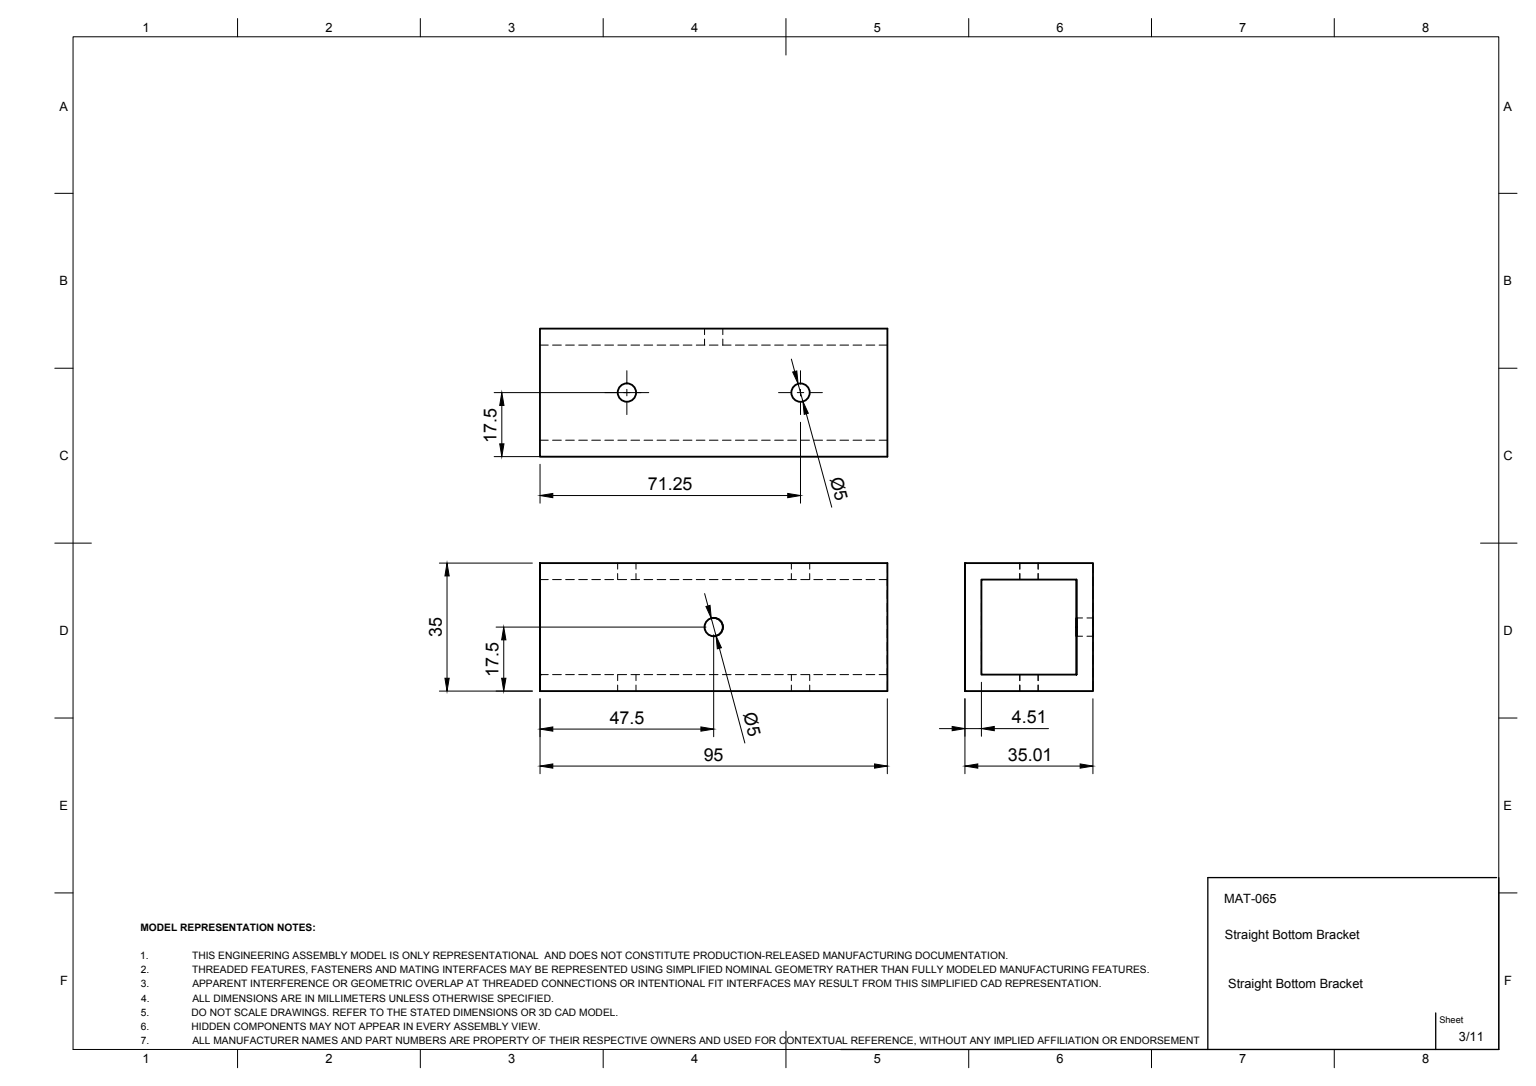
ISO-10303-21;
HEADER;
/* Generated by software containing ST-Developer
 * from STEP Tools, Inc. (www.steptools.com) 
 */

FILE_DESCRIPTION(
/* description */ (
'CAx-IF Rec.Pracs.---Representation and Presentation of Product Manufa
cturing Information (PMI)---4.0---2014-10-13'),
/* implementation_level */ '2;1');

FILE_NAME(
/* name */ 'Straight Bottom Bracket.step',
/* time_stamp */ '2026-11-15T23:28:27-08:00',
/* author */ (''),
/* organization */ (''),
/* preprocessor_version */ 'ST-DEVELOPER v20.2',
/* originating_system */ 'Autodesk Translation Framework v15.17.0.0',
/* authorisation */ '');

FILE_SCHEMA (('AUTOMOTIVE_DESIGN { 1 0 10303 214 3 1 1 }'));
ENDSEC;

DATA;
#10=MECHANICAL_DESIGN_GEOMETRIC_PRESENTATION_REPRESENTATION('',(#189),#7756);
#171=SHAPE_REPRESENTATION_RELATIONSHIP('SRR','None',#7819,#180);
#180=ADVANCED_BREP_SHAPE_REPRESENTATION('',(#198),#7747);
#189=STYLED_ITEM('',(#7873),#198);
#198=MANIFOLD_SOLID_BREP('Body1',#4626);
#207=CYLINDRICAL_SURFACE('',#4757,0.0025);
#208=CYLINDRICAL_SURFACE('',#4758,0.0025);
#209=CYLINDRICAL_SURFACE('',#4759,0.0025);
#210=CYLINDRICAL_SURFACE('',#4760,0.0025);
#211=CYLINDRICAL_SURFACE('',#4761,0.0025);
#264=CIRCLE('',#4740,0.0025);
#265=CIRCLE('',#4743,0.0025);
#266=CIRCLE('',#4744,0.0025);
#267=CIRCLE('',#4746,0.0025);
#268=CIRCLE('',#4747,0.0025);
#269=CIRCLE('',#4749,0.0025);
#270=CIRCLE('',#4750,0.0025);
#271=CIRCLE('',#4752,0.0025);
#272=CIRCLE('',#4754,0.0025);
#273=CIRCLE('',#4755,0.0025);
#378=FACE_BOUND('',#686,.T.);
#379=FACE_BOUND('',#688,.T.);
#380=FACE_BOUND('',#690,.T.);
#381=FACE_BOUND('',#693,.T.);
#382=FACE_BOUND('',#694,.T.);
#383=FACE_BOUND('',#696,.T.);
#384=FACE_BOUND('',#697,.T.);
#385=FACE_BOUND('',#699,.T.);
#386=FACE_BOUND('',#700,.T.);
#387=FACE_BOUND('',#702,.T.);
#388=FACE_BOUND('',#704,.T.);
#389=FACE_BOUND('',#705,.T.);
#452=FACE_OUTER_BOUND('',#685,.T.);
#453=FACE_OUTER_BOUND('',#687,.T.);
#454=FACE_OUTER_BOUND('',#689,.T.);
#455=FACE_OUTER_BOUND('',#691,.T.);
#456=FACE_OUTER_BOUND('',#692,.T.);
#457=FACE_OUTER_BOUND('',#695,.T.);
#458=FACE_OUTER_BOUND('',#698,.T.);
#459=FACE_OUTER_BOUND('',#701,.T.);
#460=FACE_OUTER_BOUND('',#703,.T.);
#461=FACE_OUTER_BOUND('',#706,.T.);
#462=FACE_OUTER_BOUND('',#707,.T.);
#463=FACE_OUTER_BOUND('',#708,.T.);
#464=FACE_OUTER_BOUND('',#709,.T.);
#465=FACE_OUTER_BOUND('',#710,.T.);
#466=FACE_OUTER_BOUND('',#711,.T.);
#685=EDGE_LOOP('',(#2993,#2994,#2995,#2996));
#686=EDGE_LOOP('',(#2997,#2998,#2999,#3000));
#687=EDGE_LOOP('',(#3001,#3002,#3003,#3004));
#688=EDGE_LOOP('',(#3005,#3006,#3007,#3008));
#689=EDGE_LOOP('',(#3009,#3010,#3011,#3012));
#690=EDGE_LOOP('',(#3013));
#691=EDGE_LOOP('',(#3014,#3015,#3016,#3017));
#692=EDGE_LOOP('',(#3018,#3019,#3020,#3021));
#693=EDGE_LOOP('',(#3022));
#694=EDGE_LOOP('',(#3023));
#695=EDGE_LOOP('',(#3024,#3025,#3026,#3027));
#696=EDGE_LOOP('',(#3028));
#697=EDGE_LOOP('',(#3029));
#698=EDGE_LOOP('',(#3030,#3031,#3032,#3033));
#699=EDGE_LOOP('',(#3034));
#700=EDGE_LOOP('',(#3035));
#701=EDGE_LOOP('',(#3036,#3037,#3038,#3039));
#702=EDGE_LOOP('',(#3040));
#703=EDGE_LOOP('',(#3041,#3042,#3043,#3044));
#704=EDGE_LOOP('',(#3045));
#705=EDGE_LOOP('',(#3046));
#706=EDGE_LOOP('',(#3047,#3048,#3049,#3050));
#707=EDGE_LOOP('',(#3051,#3052,#3053,#3054));
#708=EDGE_LOOP('',(#3055,#3056,#3057,#3058));
#709=EDGE_LOOP('',(#3059,#3060,#3061,#3062));
#710=EDGE_LOOP('',(#3063,#3064,#3065,#3066));
#711=EDGE_LOOP('',(#3067,#3068,#3069,#3070));
#992=LINE('',#6424,#1485);
#993=LINE('',#6426,#1486);
#994=LINE('',#6428,#1487);
#995=LINE('',#6429,#1488);
#996=LINE('',#6432,#1489);
#997=LINE('',#6434,#1490);
#998=LINE('',#6436,#1491);
#999=LINE('',#6437,#1492);
#1000=LINE('',#6441,#1493);
#1001=LINE('',#6443,#1494);
#1002=LINE('',#6445,#1495);
#1003=LINE('',#6446,#1496);
#1004=LINE('',#6449,#1497);
#1005=LINE('',#6451,#1498);
#1006=LINE('',#6453,#1499);
#1007=LINE('',#6454,#1500);
#1008=LINE('',#6456,#1501);
#1009=LINE('',#6457,#1502);
#1010=LINE('',#6461,#1503);
#1011=LINE('',#6462,#1504);
#1012=LINE('',#6474,#1505);
#1013=LINE('',#6475,#1506);
#1014=LINE('',#6481,#1507);
#1015=LINE('',#6485,#1508);
#1016=LINE('',#6492,#1509);
#1017=LINE('',#6494,#1510);
#1018=LINE('',#6496,#1511);
#1019=LINE('',#6498,#1512);
#1020=LINE('',#6500,#1513);
#1485=VECTOR('',#5138,1.);
#1486=VECTOR('',#5139,1.);
#1487=VECTOR('',#5140,1.);
#1488=VECTOR('',#5141,1.);
#1489=VECTOR('',#5142,1.);
#1490=VECTOR('',#5143,1.);
#1491=VECTOR('',#5144,1.);
#1492=VECTOR('',#5145,1.);
#1493=VECTOR('',#5148,1.);
#1494=VECTOR('',#5149,1.);
#1495=VECTOR('',#5150,1.);
#1496=VECTOR('',#5151,1.);
#1497=VECTOR('',#5152,1.);
#1498=VECTOR('',#5153,1.);
#1499=VECTOR('',#5154,1.);
#1500=VECTOR('',#5155,1.);
#1501=VECTOR('',#5158,1.);
#1502=VECTOR('',#5159,1.);
#1503=VECTOR('',#5164,1.);
#1504=VECTOR('',#5165,1.);
#1505=VECTOR('',#5180,1.);
#1506=VECTOR('',#5181,1.);
#1507=VECTOR('',#5188,1.);
#1508=VECTOR('',#5193,1.);
#1509=VECTOR('',#5202,0.0025);
#1510=VECTOR('',#5205,0.0025);
#1511=VECTOR('',#5208,0.0025);
#1512=VECTOR('',#5211,0.0025);
#1513=VECTOR('',#5214,0.0025);
#1978=VERTEX_POINT('',#6422);
#1979=VERTEX_POINT('',#6423);
#1980=VERTEX_POINT('',#6425);
#1981=VERTEX_POINT('',#6427);
#1982=VERTEX_POINT('',#6430);
#1983=VERTEX_POINT('',#6431);
#1984=VERTEX_POINT('',#6433);
#1985=VERTEX_POINT('',#6435);
#1986=VERTEX_POINT('',#6439);
#1987=VERTEX_POINT('',#6440);
#1988=VERTEX_POINT('',#6442);
#1989=VERTEX_POINT('',#6444);
#1990=VERTEX_POINT('',#6447);
#1991=VERTEX_POINT('',#6448);
#1992=VERTEX_POINT('',#6450);
#1993=VERTEX_POINT('',#6452);
#1994=VERTEX_POINT('',#6458);
#1995=VERTEX_POINT('',#6464);
#1996=VERTEX_POINT('',#6466);
#1997=VERTEX_POINT('',#6469);
#1998=VERTEX_POINT('',#6471);
#1999=VERTEX_POINT('',#6476);
#2000=VERTEX_POINT('',#6478);
#2001=VERTEX_POINT('',#6482);
#2002=VERTEX_POINT('',#6486);
#2003=VERTEX_POINT('',#6488);
#2380=EDGE_CURVE('',#1978,#1979,#992,.T.);
#2381=EDGE_CURVE('',#1980,#1979,#993,.T.);
#2382=EDGE_CURVE('',#1981,#1980,#994,.T.);
#2383=EDGE_CURVE('',#1981,#1978,#995,.T.);
#2384=EDGE_CURVE('',#1982,#1983,#996,.T.);
#2385=EDGE_CURVE('',#1983,#1984,#997,.T.);
#2386=EDGE_CURVE('',#1985,#1984,#998,.T.);
#2387=EDGE_CURVE('',#1982,#1985,#999,.T.);
#2388=EDGE_CURVE('',#1986,#1987,#1000,.T.);
#2389=EDGE_CURVE('',#1988,#1986,#1001,.T.);
#2390=EDGE_CURVE('',#1988,#1989,#1002,.T.);
#2391=EDGE_CURVE('',#1989,#1987,#1003,.T.);
#2392=EDGE_CURVE('',#1990,#1991,#1004,.T.);
#2393=EDGE_CURVE('',#1991,#1992,#1005,.T.);
#2394=EDGE_CURVE('',#1993,#1992,#1006,.T.);
#2395=EDGE_CURVE('',#1990,#1993,#1007,.T.);
#2396=EDGE_CURVE('',#1978,#1986,#1008,.T.);
#2397=EDGE_CURVE('',#1981,#1988,#1009,.T.);
#2398=EDGE_CURVE('',#1994,#1994,#264,.T.);
#2399=EDGE_CURVE('',#1979,#1987,#1010,.T.);
#2400=EDGE_CURVE('',#1980,#1989,#1011,.T.);
#2401=EDGE_CURVE('',#1995,#1995,#265,.T.);
#2402=EDGE_CURVE('',#1996,#1996,#266,.T.);
#2403=EDGE_CURVE('',#1997,#1997,#267,.T.);
#2404=EDGE_CURVE('',#1998,#1998,#268,.T.);
#2405=EDGE_CURVE('',#1991,#1983,#1012,.T.);
#2406=EDGE_CURVE('',#1992,#1982,#1013,.T.);
#2407=EDGE_CURVE('',#1999,#1999,#269,.T.);
#2408=EDGE_CURVE('',#2000,#2000,#270,.T.);
#2409=EDGE_CURVE('',#1993,#1985,#1014,.T.);
#2410=EDGE_CURVE('',#2001,#2001,#271,.T.);
#2411=EDGE_CURVE('',#1990,#1984,#1015,.T.);
#2412=EDGE_CURVE('',#2002,#2002,#272,.T.);
#2413=EDGE_CURVE('',#2003,#2003,#273,.T.);
#2414=EDGE_CURVE('',#2001,#1994,#1016,.T.);
#2415=EDGE_CURVE('',#1998,#2003,#1017,.T.);
#2416=EDGE_CURVE('',#1997,#2002,#1018,.T.);
#2417=EDGE_CURVE('',#2000,#1996,#1019,.T.);
#2418=EDGE_CURVE('',#1999,#1995,#1020,.T.);
#2993=ORIENTED_EDGE('',*,*,#2380,.T.);
#2994=ORIENTED_EDGE('',*,*,#2381,.F.);
#2995=ORIENTED_EDGE('',*,*,#2382,.F.);
#2996=ORIENTED_EDGE('',*,*,#2383,.T.);
#2997=ORIENTED_EDGE('',*,*,#2384,.T.);
#2998=ORIENTED_EDGE('',*,*,#2385,.T.);
#2999=ORIENTED_EDGE('',*,*,#2386,.F.);
#3000=ORIENTED_EDGE('',*,*,#2387,.F.);
#3001=ORIENTED_EDGE('',*,*,#2388,.F.);
#3002=ORIENTED_EDGE('',*,*,#2389,.F.);
#3003=ORIENTED_EDGE('',*,*,#2390,.T.);
#3004=ORIENTED_EDGE('',*,*,#2391,.T.);
#3005=ORIENTED_EDGE('',*,*,#2392,.T.);
#3006=ORIENTED_EDGE('',*,*,#2393,.T.);
#3007=ORIENTED_EDGE('',*,*,#2394,.F.);
#3008=ORIENTED_EDGE('',*,*,#2395,.F.);
#3009=ORIENTED_EDGE('',*,*,#2396,.F.);
#3010=ORIENTED_EDGE('',*,*,#2383,.F.);
#3011=ORIENTED_EDGE('',*,*,#2397,.T.);
#3012=ORIENTED_EDGE('',*,*,#2389,.T.);
#3013=ORIENTED_EDGE('',*,*,#2398,.F.);
#3014=ORIENTED_EDGE('',*,*,#2399,.T.);
#3015=ORIENTED_EDGE('',*,*,#2391,.F.);
#3016=ORIENTED_EDGE('',*,*,#2400,.F.);
#3017=ORIENTED_EDGE('',*,*,#2381,.T.);
#3018=ORIENTED_EDGE('',*,*,#2397,.F.);
#3019=ORIENTED_EDGE('',*,*,#2382,.T.);
#3020=ORIENTED_EDGE('',*,*,#2400,.T.);
#3021=ORIENTED_EDGE('',*,*,#2390,.F.);
#3022=ORIENTED_EDGE('',*,*,#2401,.F.);
#3023=ORIENTED_EDGE('',*,*,#2402,.F.);
#3024=ORIENTED_EDGE('',*,*,#2396,.T.);
#3025=ORIENTED_EDGE('',*,*,#2388,.T.);
#3026=ORIENTED_EDGE('',*,*,#2399,.F.);
#3027=ORIENTED_EDGE('',*,*,#2380,.F.);
#3028=ORIENTED_EDGE('',*,*,#2403,.T.);
#3029=ORIENTED_EDGE('',*,*,#2404,.T.);
#3030=ORIENTED_EDGE('',*,*,#2405,.T.);
#3031=ORIENTED_EDGE('',*,*,#2384,.F.);
#3032=ORIENTED_EDGE('',*,*,#2406,.F.);
#3033=ORIENTED_EDGE('',*,*,#2393,.F.);
#3034=ORIENTED_EDGE('',*,*,#2407,.F.);
#3035=ORIENTED_EDGE('',*,*,#2408,.F.);
#3036=ORIENTED_EDGE('',*,*,#2394,.T.);
#3037=ORIENTED_EDGE('',*,*,#2406,.T.);
#3038=ORIENTED_EDGE('',*,*,#2387,.T.);
#3039=ORIENTED_EDGE('',*,*,#2409,.F.);
#3040=ORIENTED_EDGE('',*,*,#2410,.T.);
#3041=ORIENTED_EDGE('',*,*,#2395,.T.);
#3042=ORIENTED_EDGE('',*,*,#2409,.T.);
#3043=ORIENTED_EDGE('',*,*,#2386,.T.);
#3044=ORIENTED_EDGE('',*,*,#2411,.F.);
#3045=ORIENTED_EDGE('',*,*,#2412,.T.);
#3046=ORIENTED_EDGE('',*,*,#2413,.T.);
#3047=ORIENTED_EDGE('',*,*,#2411,.T.);
#3048=ORIENTED_EDGE('',*,*,#2385,.F.);
#3049=ORIENTED_EDGE('',*,*,#2405,.F.);
#3050=ORIENTED_EDGE('',*,*,#2392,.F.);
#3051=ORIENTED_EDGE('',*,*,#2410,.F.);
#3052=ORIENTED_EDGE('',*,*,#2414,.T.);
#3053=ORIENTED_EDGE('',*,*,#2398,.T.);
#3054=ORIENTED_EDGE('',*,*,#2414,.F.);
#3055=ORIENTED_EDGE('',*,*,#2404,.F.);
#3056=ORIENTED_EDGE('',*,*,#2415,.T.);
#3057=ORIENTED_EDGE('',*,*,#2413,.F.);
#3058=ORIENTED_EDGE('',*,*,#2415,.F.);
#3059=ORIENTED_EDGE('',*,*,#2403,.F.);
#3060=ORIENTED_EDGE('',*,*,#2416,.T.);
#3061=ORIENTED_EDGE('',*,*,#2412,.F.);
#3062=ORIENTED_EDGE('',*,*,#2416,.F.);
#3063=ORIENTED_EDGE('',*,*,#2408,.T.);
#3064=ORIENTED_EDGE('',*,*,#2417,.T.);
#3065=ORIENTED_EDGE('',*,*,#2402,.T.);
#3066=ORIENTED_EDGE('',*,*,#2417,.F.);
#3067=ORIENTED_EDGE('',*,*,#2407,.T.);
#3068=ORIENTED_EDGE('',*,*,#2418,.T.);
#3069=ORIENTED_EDGE('',*,*,#2401,.T.);
#3070=ORIENTED_EDGE('',*,*,#2418,.F.);
#4219=PLANE('',#4737);
#4220=PLANE('',#4738);
#4221=PLANE('',#4739);
#4222=PLANE('',#4741);
#4223=PLANE('',#4742);
#4224=PLANE('',#4745);
#4225=PLANE('',#4748);
#4226=PLANE('',#4751);
#4227=PLANE('',#4753);
#4228=PLANE('',#4756);
#4393=ADVANCED_FACE('',(#452,#378),#4219,.F.);
#4394=ADVANCED_FACE('',(#453,#379),#4220,.T.);
#4395=ADVANCED_FACE('',(#454,#380),#4221,.T.);
#4396=ADVANCED_FACE('',(#455),#4222,.F.);
#4397=ADVANCED_FACE('',(#456,#381,#382),#4223,.T.);
#4398=ADVANCED_FACE('',(#457,#383,#384),#4224,.F.);
#4399=ADVANCED_FACE('',(#458,#385,#386),#4225,.T.);
#4400=ADVANCED_FACE('',(#459,#387),#4226,.F.);
#4401=ADVANCED_FACE('',(#460,#388,#389),#4227,.F.);
#4402=ADVANCED_FACE('',(#461),#4228,.T.);
#4403=ADVANCED_FACE('',(#462),#207,.F.);
#4404=ADVANCED_FACE('',(#463),#208,.F.);
#4405=ADVANCED_FACE('',(#464),#209,.F.);
#4406=ADVANCED_FACE('',(#465),#210,.F.);
#4407=ADVANCED_FACE('',(#466),#211,.F.);
#4626=CLOSED_SHELL('',(#4393,#4394,#4395,#4396,#4397,#4398,#4399,#4400,
#4401,#4402,#4403,#4404,#4405,#4406,#4407));
#4736=AXIS2_PLACEMENT_3D('',#6420,#5134,#5135);
#4737=AXIS2_PLACEMENT_3D('',#6421,#5136,#5137);
#4738=AXIS2_PLACEMENT_3D('',#6438,#5146,#5147);
#4739=AXIS2_PLACEMENT_3D('',#6455,#5156,#5157);
#4740=AXIS2_PLACEMENT_3D('',#6459,#5160,#5161);
#4741=AXIS2_PLACEMENT_3D('',#6460,#5162,#5163);
#4742=AXIS2_PLACEMENT_3D('',#6463,#5166,#5167);
#4743=AXIS2_PLACEMENT_3D('',#6465,#5168,#5169);
#4744=AXIS2_PLACEMENT_3D('',#6467,#5170,#5171);
#4745=AXIS2_PLACEMENT_3D('',#6468,#5172,#5173);
#4746=AXIS2_PLACEMENT_3D('',#6470,#5174,#5175);
#4747=AXIS2_PLACEMENT_3D('',#6472,#5176,#5177);
#4748=AXIS2_PLACEMENT_3D('',#6473,#5178,#5179);
#4749=AXIS2_PLACEMENT_3D('',#6477,#5182,#5183);
#4750=AXIS2_PLACEMENT_3D('',#6479,#5184,#5185);
#4751=AXIS2_PLACEMENT_3D('',#6480,#5186,#5187);
#4752=AXIS2_PLACEMENT_3D('',#6483,#5189,#5190);
#4753=AXIS2_PLACEMENT_3D('',#6484,#5191,#5192);
#4754=AXIS2_PLACEMENT_3D('',#6487,#5194,#5195);
#4755=AXIS2_PLACEMENT_3D('',#6489,#5196,#5197);
#4756=AXIS2_PLACEMENT_3D('',#6490,#5198,#5199);
#4757=AXIS2_PLACEMENT_3D('',#6491,#5200,#5201);
#4758=AXIS2_PLACEMENT_3D('',#6493,#5203,#5204);
#4759=AXIS2_PLACEMENT_3D('',#6495,#5206,#5207);
#4760=AXIS2_PLACEMENT_3D('',#6497,#5209,#5210);
#4761=AXIS2_PLACEMENT_3D('',#6499,#5212,#5213);
#5134=DIRECTION('axis',(0.,0.,1.));
#5135=DIRECTION('refdir',(1.,0.,0.));
#5136=DIRECTION('center_axis',(1.,0.,0.));
#5137=DIRECTION('ref_axis',(0.,0.,-1.));
#5138=DIRECTION('',(0.,-1.,0.));
#5139=DIRECTION('',(0.,0.,-1.));
#5140=DIRECTION('',(0.,-1.,0.));
#5141=DIRECTION('',(0.,0.,-1.));
#5142=DIRECTION('',(0.,-1.,0.));
#5143=DIRECTION('',(0.,0.,-1.));
#5144=DIRECTION('',(0.,-1.,0.));
#5145=DIRECTION('',(0.,-6.67201336914157E-17,-1.));
#5146=DIRECTION('center_axis',(1.,0.,0.));
#5147=DIRECTION('ref_axis',(0.,0.,-1.));
#5148=DIRECTION('',(0.,-1.,0.));
#5149=DIRECTION('',(0.,0.,-1.));
#5150=DIRECTION('',(0.,-1.,0.));
#5151=DIRECTION('',(0.,0.,-1.));
#5152=DIRECTION('',(0.,0.,1.));
#5153=DIRECTION('',(0.,1.,0.));
#5154=DIRECTION('',(0.,6.67201336914157E-17,1.));
#5155=DIRECTION('',(0.,1.,0.));
#5156=DIRECTION('center_axis',(-1.82602471155453E-16,1.,0.));
#5157=DIRECTION('ref_axis',(-1.,-1.82602471155453E-16,0.));
#5158=DIRECTION('',(1.,1.82602471155453E-16,0.));
#5159=DIRECTION('',(1.,1.82602471155453E-16,0.));
#5160=DIRECTION('center_axis',(-1.82602471155453E-16,1.,0.));
#5161=DIRECTION('ref_axis',(-1.,-1.82602471155453E-16,0.));
#5162=DIRECTION('center_axis',(-2.19122965386544E-16,1.,0.));
#5163=DIRECTION('ref_axis',(-1.,-2.19122965386544E-16,0.));
#5164=DIRECTION('',(1.,2.19122965386544E-16,0.));
#5165=DIRECTION('',(1.,2.19122965386544E-16,0.));
#5166=DIRECTION('center_axis',(0.,0.,1.));
#5167=DIRECTION('ref_axis',(1.,0.,0.));
#5168=DIRECTION('center_axis',(0.,0.,1.));
#5169=DIRECTION('ref_axis',(1.,0.,0.));
#5170=DIRECTION('center_axis',(0.,0.,1.));
#5171=DIRECTION('ref_axis',(1.,0.,0.));
#5172=DIRECTION('center_axis',(0.,0.,1.));
#5173=DIRECTION('ref_axis',(1.,0.,0.));
#5174=DIRECTION('center_axis',(0.,0.,1.));
#5175=DIRECTION('ref_axis',(1.,0.,0.));
#5176=DIRECTION('center_axis',(0.,0.,1.));
#5177=DIRECTION('ref_axis',(1.,0.,0.));
#5178=DIRECTION('center_axis',(0.,0.,-1.));
#5179=DIRECTION('ref_axis',(-1.,0.,0.));
#5180=DIRECTION('',(-1.,0.,0.));
#5181=DIRECTION('',(-1.,0.,0.));
#5182=DIRECTION('center_axis',(0.,0.,-1.));
#5183=DIRECTION('ref_axis',(-1.,0.,0.));
#5184=DIRECTION('center_axis',(0.,0.,-1.));
#5185=DIRECTION('ref_axis',(-1.,0.,0.));
#5186=DIRECTION('center_axis',(0.,1.,-6.67201336914157E-17));
#5187=DIRECTION('ref_axis',(0.,6.67201336914157E-17,1.));
#5188=DIRECTION('',(-1.,0.,0.));
#5189=DIRECTION('center_axis',(0.,1.,-6.67201336914157E-17));
#5190=DIRECTION('ref_axis',(0.,6.67201336914157E-17,1.));
#5191=DIRECTION('center_axis',(0.,0.,-1.));
#5192=DIRECTION('ref_axis',(-1.,0.,0.));
#5193=DIRECTION('',(-1.,0.,0.));
#5194=DIRECTION('center_axis',(0.,0.,-1.));
#5195=DIRECTION('ref_axis',(-1.,0.,0.));
#5196=DIRECTION('center_axis',(0.,0.,-1.));
#5197=DIRECTION('ref_axis',(-1.,0.,0.));
#5198=DIRECTION('center_axis',(0.,1.,0.));
#5199=DIRECTION('ref_axis',(0.,0.,1.));
#5200=DIRECTION('center_axis',(-1.82602471155453E-16,1.,0.));
#5201=DIRECTION('ref_axis',(-1.,-1.82602471155453E-16,0.));
#5202=DIRECTION('',(-1.82602471155453E-16,1.,0.));
#5203=DIRECTION('center_axis',(0.,0.,1.));
#5204=DIRECTION('ref_axis',(1.,0.,0.));
#5205=DIRECTION('',(0.,0.,1.));
#5206=DIRECTION('center_axis',(0.,0.,1.));
#5207=DIRECTION('ref_axis',(1.,0.,0.));
#5208=DIRECTION('',(0.,0.,1.));
#5209=DIRECTION('center_axis',(0.,0.,1.));
#5210=DIRECTION('ref_axis',(1.,0.,0.));
#5211=DIRECTION('',(0.,0.,1.));
#5212=DIRECTION('center_axis',(0.,0.,1.));
#5213=DIRECTION('ref_axis',(1.,0.,0.));
#5214=DIRECTION('',(0.,0.,1.));
#6420=CARTESIAN_POINT('',(0.,0.,0.));
#6421=CARTESIAN_POINT('Origin',(-0.0475,-1.04083408558608E-17,0.035));
#6422=CARTESIAN_POINT('',(-0.0475,0.0175,0.));
#6423=CARTESIAN_POINT('',(-0.0475,-0.0175,0.));
#6424=CARTESIAN_POINT('',(-0.0475,-1.04083408558608E-17,0.));
#6425=CARTESIAN_POINT('',(-0.0475,-0.0175,0.035));
#6426=CARTESIAN_POINT('',(-0.0475,-0.0175,0.035));
#6427=CARTESIAN_POINT('',(-0.0475,0.0175,0.035));
#6428=CARTESIAN_POINT('',(-0.0475,-1.04083408558608E-17,0.035));
#6429=CARTESIAN_POINT('',(-0.0475,0.0175,0.035));
#6430=CARTESIAN_POINT('',(-0.0475,0.013,0.0305));
#6431=CARTESIAN_POINT('',(-0.0475,-0.013,0.0305));
#6432=CARTESIAN_POINT('',(-0.0475,-1.04083408558608E-17,0.0305));
#6433=CARTESIAN_POINT('',(-0.0475,-0.013,0.0045));
#6434=CARTESIAN_POINT('',(-0.0475,-0.013,0.0175));
#6435=CARTESIAN_POINT('',(-0.0475,0.013,0.0045));
#6436=CARTESIAN_POINT('',(-0.0475,-1.21430643318376E-17,0.0045));
#6437=CARTESIAN_POINT('',(-0.0475,0.013,0.0175));
#6438=CARTESIAN_POINT('Origin',(0.0475,6.93889390390723E-18,0.035));
#6439=CARTESIAN_POINT('',(0.0475,0.0175,0.));
#6440=CARTESIAN_POINT('',(0.0475,-0.0175,0.));
#6441=CARTESIAN_POINT('',(0.0475,6.93889390390723E-18,0.));
#6442=CARTESIAN_POINT('',(0.0475,0.0175,0.035));
#6443=CARTESIAN_POINT('',(0.0475,0.0175,0.035));
#6444=CARTESIAN_POINT('',(0.0475,-0.0175,0.035));
#6445=CARTESIAN_POINT('',(0.0475,6.93889390390723E-18,0.035));
#6446=CARTESIAN_POINT('',(0.0475,-0.0175,0.035));
#6447=CARTESIAN_POINT('',(0.0475,-0.013,0.0045));
#6448=CARTESIAN_POINT('',(0.0475,-0.013,0.0305));
#6449=CARTESIAN_POINT('',(0.0475,-0.013,0.035));
#6450=CARTESIAN_POINT('',(0.0475,0.013,0.0305));
#6451=CARTESIAN_POINT('',(0.0475,6.93889390390723E-18,0.0305));
#6452=CARTESIAN_POINT('',(0.0475,0.013,0.0045));
#6453=CARTESIAN_POINT('',(0.0475,0.013,0.035));
#6454=CARTESIAN_POINT('',(0.0475,6.93889390390723E-18,0.0045));
#6455=CARTESIAN_POINT('Origin',(6.93889390390723E-18,0.0175,0.035));
#6456=CARTESIAN_POINT('',(6.93889390390723E-18,0.0175,0.));
#6457=CARTESIAN_POINT('',(6.93889390390723E-18,0.0175,0.035));
#6458=CARTESIAN_POINT('',(0.0025,0.0175,0.0175));
#6459=CARTESIAN_POINT('Origin',(-3.46944695195361E-18,0.0175,0.0175));
#6460=CARTESIAN_POINT('Origin',(6.93889390390723E-18,-0.0175,0.035));
#6461=CARTESIAN_POINT('',(6.93889390390723E-18,-0.0175,0.));
#6462=CARTESIAN_POINT('',(6.93889390390723E-18,-0.0175,0.035));
#6463=CARTESIAN_POINT('Origin',(6.93889390390723E-18,0.,0.035));
#6464=CARTESIAN_POINT('',(-0.02625,-1.53080849893419E-19,0.035));
#6465=CARTESIAN_POINT('Origin',(-0.02375,1.53080849893419E-19,0.035));
#6466=CARTESIAN_POINT('',(0.02125,-3.08148791101958E-34,0.035));
#6467=CARTESIAN_POINT('Origin',(0.02375,3.06161699786838E-19,0.035));
#6468=CARTESIAN_POINT('Origin',(6.93889390390723E-18,0.,0.));
#6469=CARTESIAN_POINT('',(-0.02625,-1.53080849893419E-19,0.));
#6470=CARTESIAN_POINT('Origin',(-0.02375,1.53080849893419E-19,0.));
#6471=CARTESIAN_POINT('',(0.02125,-3.08148791101958E-34,0.));
#6472=CARTESIAN_POINT('Origin',(0.02375,3.06161699786838E-19,0.));
#6473=CARTESIAN_POINT('Origin',(0.0525,-1.04083408558608E-17,0.0305));
#6474=CARTESIAN_POINT('',(0.0525,-0.013,0.0305));
#6475=CARTESIAN_POINT('',(0.0525,0.013,0.0305));
#6476=CARTESIAN_POINT('',(-0.02625,1.53080849893419E-19,0.0305));
#6477=CARTESIAN_POINT('Origin',(-0.02375,1.53080849893419E-19,0.0305));
#6478=CARTESIAN_POINT('',(0.02125,3.06161699786838E-19,0.0305));
#6479=CARTESIAN_POINT('Origin',(0.02375,3.06161699786838E-19,0.0305));
#6480=CARTESIAN_POINT('Origin',(0.0525,0.013,0.0175));
#6481=CARTESIAN_POINT('',(0.0525,0.013,0.0045));
#6482=CARTESIAN_POINT('',(0.0025,0.013,0.0175));
#6483=CARTESIAN_POINT('Origin',(-2.64773583175407E-18,0.013,0.0175));
#6484=CARTESIAN_POINT('Origin',(0.0525,-1.21430643318376E-17,0.0045));
#6485=CARTESIAN_POINT('',(0.0525,-0.013,0.0045));
#6486=CARTESIAN_POINT('',(-0.02625,1.53080849893419E-19,0.0045));
#6487=CARTESIAN_POINT('Origin',(-0.02375,1.53080849893419E-19,0.0045));
#6488=CARTESIAN_POINT('',(0.02125,3.06161699786838E-19,0.0045));
#6489=CARTESIAN_POINT('Origin',(0.02375,3.06161699786838E-19,0.0045));
#6490=CARTESIAN_POINT('Origin',(0.0525,-0.013,0.0175));
#6491=CARTESIAN_POINT('Origin',(-1.64342224039908E-18,0.0075,0.0175));
#6492=CARTESIAN_POINT('',(0.0025,0.0075,0.0175));
#6493=CARTESIAN_POINT('Origin',(0.02375,3.06161699786838E-19,-0.005));
#6494=CARTESIAN_POINT('',(0.02125,-3.08148791101958E-34,-0.005));
#6495=CARTESIAN_POINT('Origin',(-0.02375,1.53080849893419E-19,-0.005));
#6496=CARTESIAN_POINT('',(-0.02625,-1.53080849893419E-19,-0.005));
#6497=CARTESIAN_POINT('Origin',(0.02375,3.06161699786838E-19,-0.005));
#6498=CARTESIAN_POINT('',(0.02125,-3.08148791101958E-34,-0.005));
#6499=CARTESIAN_POINT('Origin',(-0.02375,1.53080849893419E-19,-0.005));
#6500=CARTESIAN_POINT('',(-0.02625,-1.53080849893419E-19,-0.005));
#7736=UNCERTAINTY_MEASURE_WITH_UNIT(LENGTH_MEASURE(1.E-5),#7757,
'DISTANCE_ACCURACY_VALUE',
'Maximum model space distance between geometric entities at asserted c
onnectivities');
#7745=UNCERTAINTY_MEASURE_WITH_UNIT(LENGTH_MEASURE(1.E-5),#7757,
'DISTANCE_ACCURACY_VALUE',
'Maximum model space distance between geometric entities at asserted c
onnectivities');
#7747=(
GEOMETRIC_REPRESENTATION_CONTEXT(3)
GLOBAL_UNCERTAINTY_ASSIGNED_CONTEXT((#7736))
GLOBAL_UNIT_ASSIGNED_CONTEXT((#7757,#7758,#7759))
REPRESENTATION_CONTEXT('','3D')
);
#7756=(
GEOMETRIC_REPRESENTATION_CONTEXT(3)
GLOBAL_UNCERTAINTY_ASSIGNED_CONTEXT((#7745))
GLOBAL_UNIT_ASSIGNED_CONTEXT((#7757,#7758,#7759))
REPRESENTATION_CONTEXT('','3D')
);
#7757=(
LENGTH_UNIT()
NAMED_UNIT(*)
SI_UNIT($,.METRE.)
);
#7758=(
NAMED_UNIT(*)
PLANE_ANGLE_UNIT()
SI_UNIT($,.RADIAN.)
);
#7759=(
NAMED_UNIT(*)
SI_UNIT($,.STERADIAN.)
SOLID_ANGLE_UNIT()
);
#7761=SHAPE_DEFINITION_REPRESENTATION(#7771,#7819);
#7771=PRODUCT_DEFINITION_SHAPE('',$,#7830);
#7819=SHAPE_REPRESENTATION('',(#4736),#7747);
#7828=PRODUCT_DEFINITION_CONTEXT('part definition',#7860,'design');
#7830=PRODUCT_DEFINITION('Straight Bottom Bracket',
'Straight Bottom Bracket',#7840,#7828);
#7840=PRODUCT_DEFINITION_FORMATION('',$,#7863);
#7860=APPLICATION_CONTEXT(
'Core Data for Automotive Mechanical Design Process');
#7861=PRODUCT_CONTEXT('part definition',#7860,'mechanical');
#7863=PRODUCT('Straight Bottom Bracket','Straight Bottom Bracket',
'LEGAL AND USAGE DISCLAIMER: this Data/Model is provided \X2\201C\X0\A
S IS\X2\201D\X0\ for informational and representational only. It is a 
geometric approximation and is NOT engineered, certified, or guarantee
d for dimensional accuracy, exact tolerances, or production-level prec
ision. Vendor disclaims all implied warranties including fitness for a
 particular purpose. DO NOT USE FOR DIRECT PHYSICAL MANUFACTURING, AUT
OMATED PRODUCTION, OR SAFETY-CRITICAL SYSTEMS without independent engi
neering verification and resolution of any design discrepancies.',(#7861));
#7873=PRESENTATION_STYLE_ASSIGNMENT((#7880));
#7880=SURFACE_STYLE_USAGE(.BOTH.,#7887);
#7887=SURFACE_SIDE_STYLE('',(#7894));
#7894=SURFACE_STYLE_FILL_AREA(#7901);
#7901=FILL_AREA_STYLE('Opaque(246,246,243)',(#7908));
#7908=FILL_AREA_STYLE_COLOUR('Opaque(246,246,243)',#7915);
#7915=COLOUR_RGB('Opaque(246,246,243)',0.964705882352941,0.964705882352941,
0.952941176470588);
ENDSEC;
END-ISO-10303-21;
